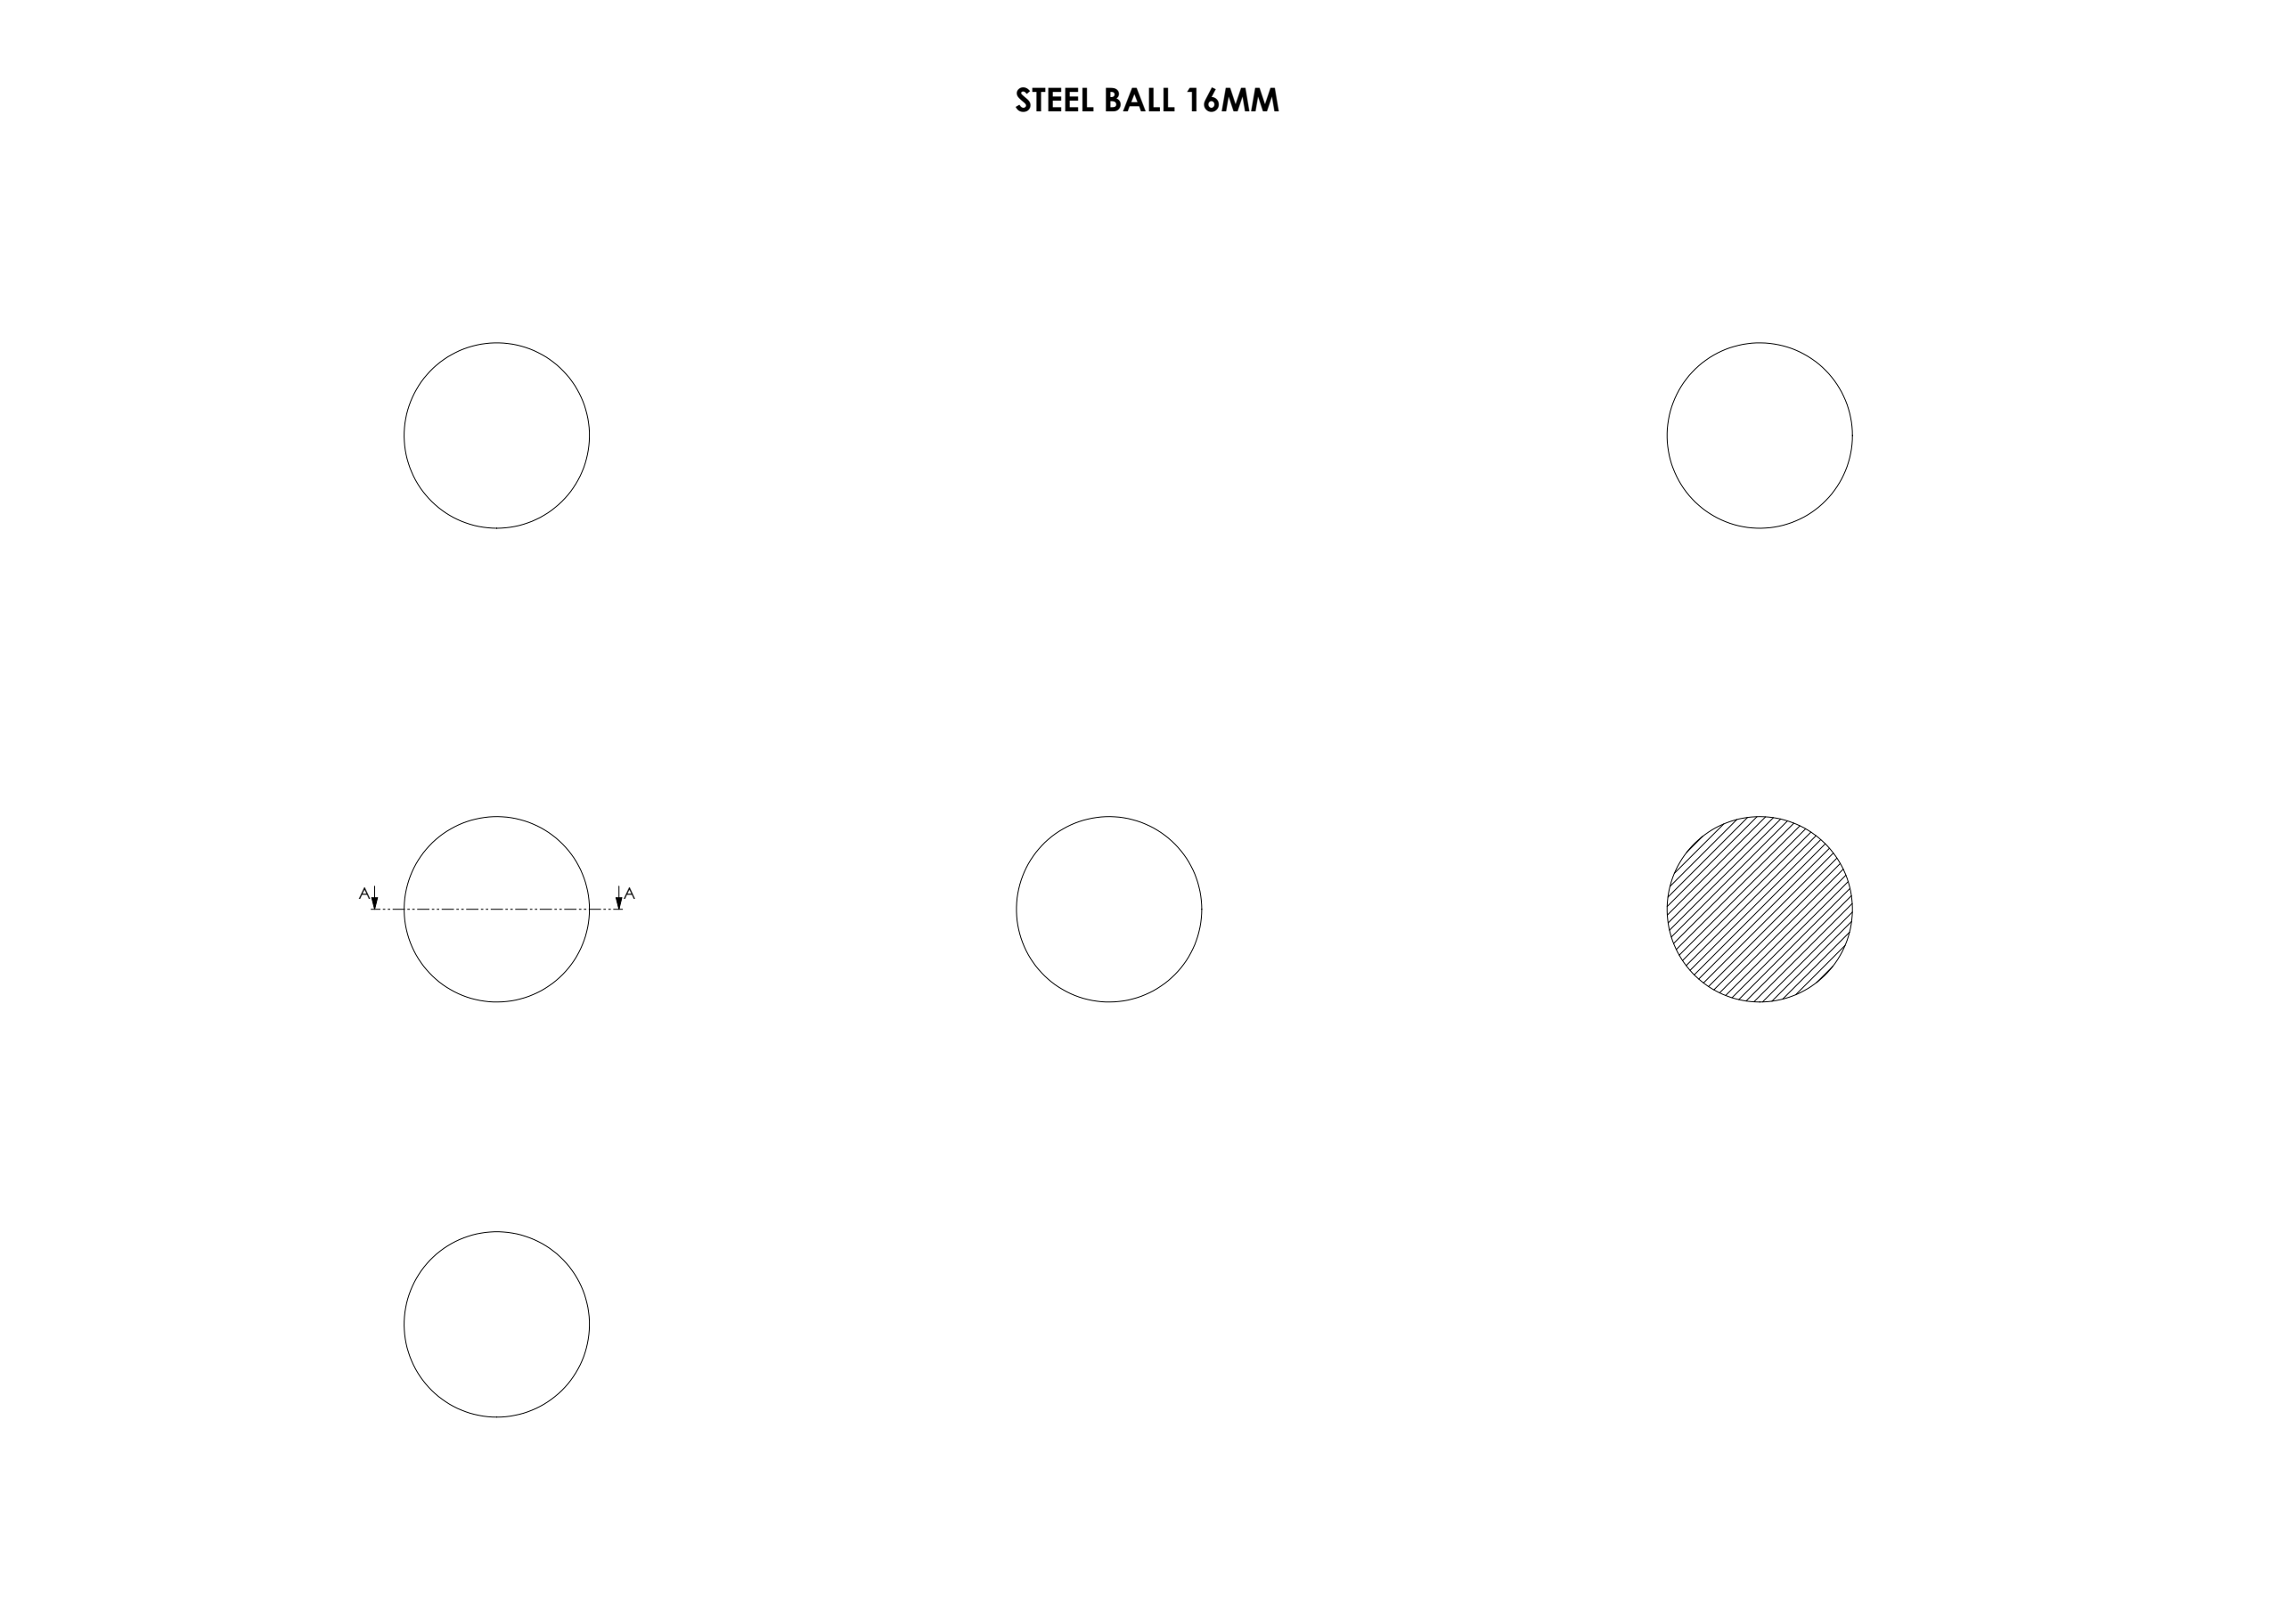
ISO-10303-21;
HEADER;
/* Generated by software containing ST-Developer
 * from STEP Tools, Inc. (www.steptools.com) 
 */

FILE_DESCRIPTION(
/* description */ (''),
/* implementation_level */ '2;1');

FILE_NAME(
/* name */ '06_Steel_Ball_16mm.step',
/* time_stamp */ '2026-10-11T12:57:03-07:00',
/* author */ (''),
/* organization */ (''),
/* preprocessor_version */ 'ST-DEVELOPER v20.2',
/* originating_system */ 'Autodesk Translation Framework v15.15.0.0',
/* authorisation */ '');

FILE_SCHEMA (('AUTOMOTIVE_DESIGN { 1 0 10303 214 3 1 1 }'));
ENDSEC;

DATA;
#10=MECHANICAL_DESIGN_GEOMETRIC_PRESENTATION_REPRESENTATION('',(#261),#90374);
#227=SHAPE_REPRESENTATION_RELATIONSHIP('SRR','None',#90446,#244);
#244=ADVANCED_BREP_SHAPE_REPRESENTATION('',(#278),#90362);
#261=STYLED_ITEM('',(#90673),#278);
#278=MANIFOLD_SOLID_BREP('Body1',#40350);
#566=SPHERICAL_SURFACE('',#43793,8.);
#3805=FACE_OUTER_BOUND('',#6228,.T.);
#6228=EDGE_LOOP('',(#33265,#33266));
#8678=CIRCLE('',#43794,8.);
#17772=VERTEX_POINT('',#81228);
#17773=VERTEX_POINT('',#81229);
#23144=EDGE_CURVE('',#17772,#17773,#8678,.T.);
#33265=ORIENTED_EDGE('',*,*,#23144,.T.);
#33266=ORIENTED_EDGE('',*,*,#23144,.F.);
#39608=ADVANCED_FACE('',(#3805),#566,.T.);
#40350=CLOSED_SHELL('',(#39608));
#43792=AXIS2_PLACEMENT_3D('',#81226,#53263,#53264);
#43793=AXIS2_PLACEMENT_3D('',#81227,#53265,#53266);
#43794=AXIS2_PLACEMENT_3D('',#81230,#53267,#53268);
#53263=DIRECTION('axis',(0.,0.,1.));
#53264=DIRECTION('refdir',(1.,0.,0.));
#53265=DIRECTION('center_axis',(6.12323399573677E-17,0.,1.));
#53266=DIRECTION('ref_axis',(1.,0.,0.));
#53267=DIRECTION('center_axis',(1.22464679914735E-16,-1.,0.));
#53268=DIRECTION('ref_axis',(-1.,-1.22464679914735E-16,0.));
#81226=CARTESIAN_POINT('',(0.,0.,0.));
#81227=CARTESIAN_POINT('Origin',(0.,0.,0.));
#81228=CARTESIAN_POINT('',(-4.89858719658941E-16,-5.99903913064743E-32,
8.));
#81229=CARTESIAN_POINT('',(-4.89858719658941E-16,-5.99903913064743E-32,
-8.));
#81230=CARTESIAN_POINT('Origin',(0.,0.,0.));
#90343=UNCERTAINTY_MEASURE_WITH_UNIT(LENGTH_MEASURE(0.01),#90375,
'DISTANCE_ACCURACY_VALUE',
'Maximum model space distance between geometric entities at asserted c
onnectivities');
#90355=UNCERTAINTY_MEASURE_WITH_UNIT(LENGTH_MEASURE(0.01),#90375,
'DISTANCE_ACCURACY_VALUE',
'Maximum model space distance between geometric entities at asserted c
onnectivities');
#90362=(
GEOMETRIC_REPRESENTATION_CONTEXT(3)
GLOBAL_UNCERTAINTY_ASSIGNED_CONTEXT((#90343))
GLOBAL_UNIT_ASSIGNED_CONTEXT((#90375,#90377,#90378))
REPRESENTATION_CONTEXT('','3D')
);
#90374=(
GEOMETRIC_REPRESENTATION_CONTEXT(3)
GLOBAL_UNCERTAINTY_ASSIGNED_CONTEXT((#90355))
GLOBAL_UNIT_ASSIGNED_CONTEXT((#90375,#90377,#90378))
REPRESENTATION_CONTEXT('','3D')
);
#90375=(
LENGTH_UNIT()
NAMED_UNIT(*)
SI_UNIT(.MILLI.,.METRE.)
);
#90377=(
NAMED_UNIT(*)
PLANE_ANGLE_UNIT()
SI_UNIT($,.RADIAN.)
);
#90378=(
NAMED_UNIT(*)
SI_UNIT($,.STERADIAN.)
SOLID_ANGLE_UNIT()
);
#90385=SHAPE_DEFINITION_REPRESENTATION(#90403,#90446);
#90403=PRODUCT_DEFINITION_SHAPE('',$,#90465);
#90446=SHAPE_REPRESENTATION('',(#43792),#90362);
#90458=PRODUCT_DEFINITION_CONTEXT('part definition',#90514,'design');
#90465=PRODUCT_DEFINITION('2026-10-11-12-53-10-468',
'06_Steel_Ball_16mm',#90483,#90458);
#90483=PRODUCT_DEFINITION_FORMATION('',$,#90522);
#90514=APPLICATION_CONTEXT(
'Core Data for Automotive Mechanical Design Process');
#90515=PRODUCT_CONTEXT('part definition',#90514,'mechanical');
#90522=PRODUCT('2026-10-11-12-53-10-468','06_Steel_Ball_16mm',$,(#90515));
#90667=COLOUR_RGB('Light Blue',0.38,0.62,0.78);
#90668=FILL_AREA_STYLE_COLOUR('',#90667);
#90669=FILL_AREA_STYLE('',(#90668));
#90670=SURFACE_STYLE_FILL_AREA(#90669);
#90671=SURFACE_SIDE_STYLE('',(#90670));
#90672=SURFACE_STYLE_USAGE(.BOTH.,#90671);
#90673=PRESENTATION_STYLE_ASSIGNMENT((#90672));
ENDSEC;
END-ISO-10303-21;
